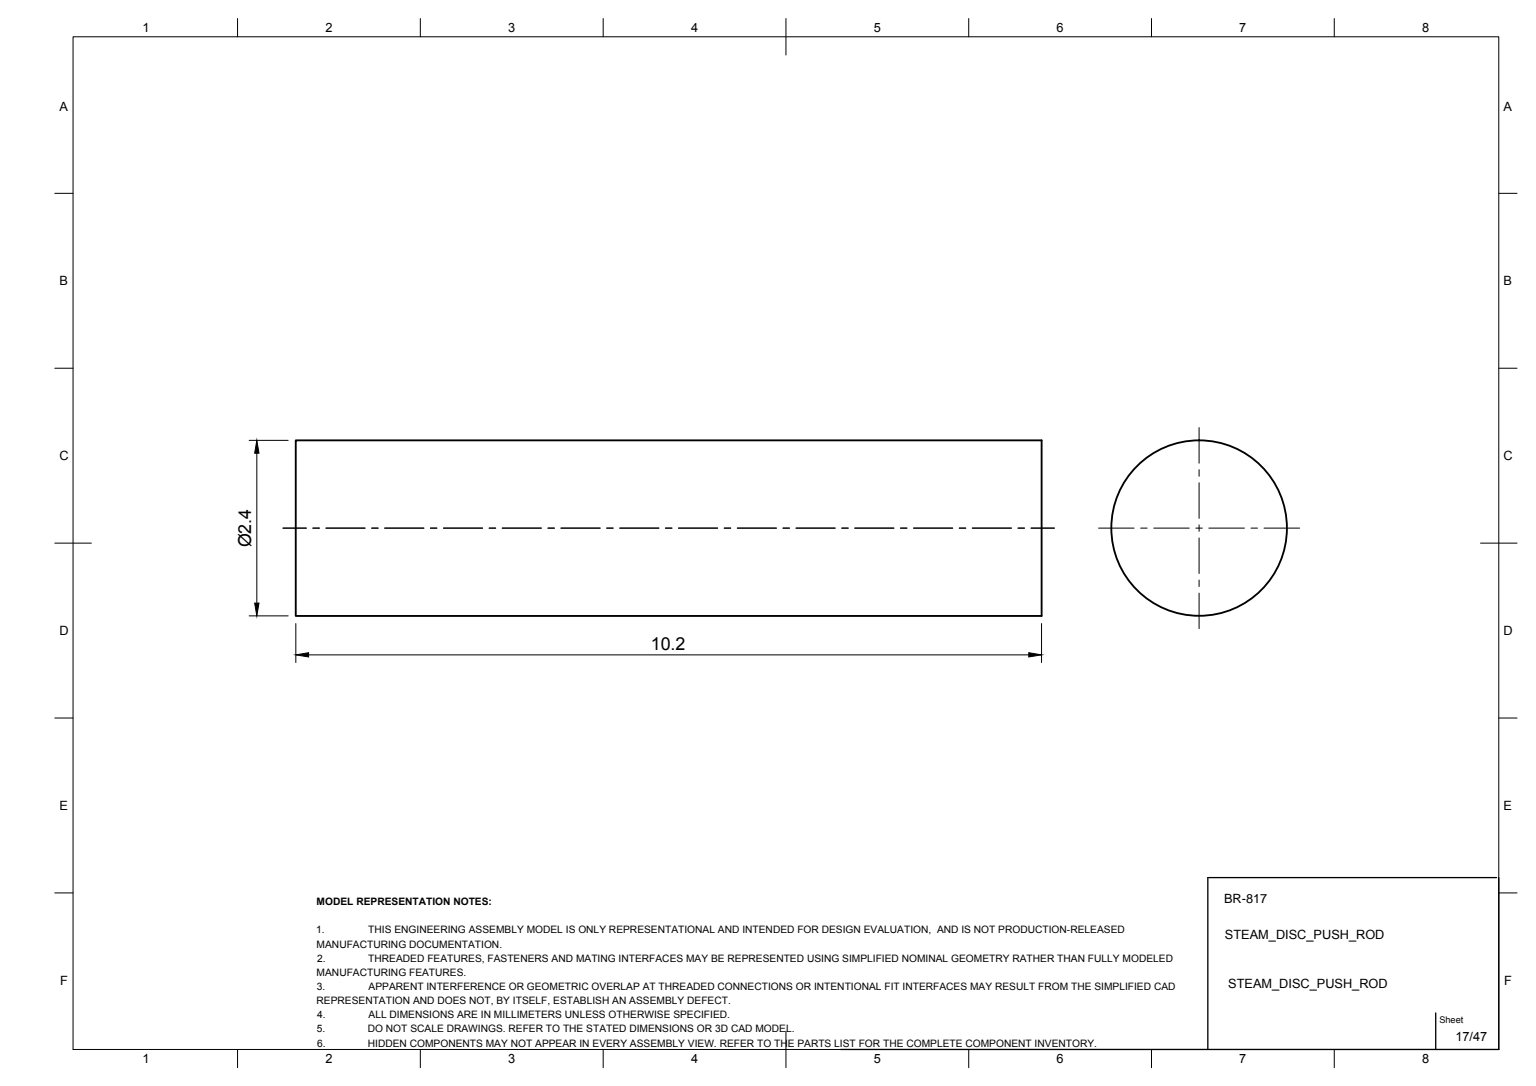
ISO-10303-21;
HEADER;
FILE_DESCRIPTION((''),'2;1');
FILE_NAME('STEAM_DISC_PUSH_ROD.step','2026-10-01T22:07:29-07:00',(''),(''),'','','');
FILE_SCHEMA (('AUTOMOTIVE_DESIGN { 1 0 10303 214 3 1 1 }'));
ENDSEC;
DATA;
#10=MECHANICAL_DESIGN_GEOMETRIC_PRESENTATION_REPRESENTATION('',(#551),#15484);
#481=SHAPE_REPRESENTATION_RELATIONSHIP('SRR','None',#15630,#516) ;
#516=ADVANCED_BREP_SHAPE_REPRESENTATION('',(#593),#15454) ;
#551=STYLED_ITEM('',(#15832),#593) ;
#593=MANIFOLD_SOLID_BREP('STEAM_DISC_PUSH_ROD',#8260) ;
#662=CYLINDRICAL_SURFACE('',#8894,0.12) ;
#958=CIRCLE('',#8895,0.12) ;
#959=CIRCLE('',#8896,0.12) ;
#1485=FACE_OUTER_BOUND('',#2028,.T.) ;
#1486=FACE_OUTER_BOUND('',#2029,.T.) ;
#1487=FACE_OUTER_BOUND('',#2030,.T.) ;
#2028=EDGE_LOOP('',(#5773,#5774,#5775,#5776)) ;
#2029=EDGE_LOOP('',(#5777)) ;
#2030=EDGE_LOOP('',(#5778)) ;
#2617=LINE('',#13445,#3091) ;
#3091=VECTOR('',#10530,0.12) ;
#3555=VERTEX_POINT('',#13442) ;
#3556=VERTEX_POINT('',#13444) ;
#4391=EDGE_CURVE('',#3555,#3555,#958,.T.) ;
#4392=EDGE_CURVE('',#3555,#3556,#2617,.T.) ;
#4393=EDGE_CURVE('',#3556,#3556,#959,.T.) ;
#5773=ORIENTED_EDGE('',*,*,#4391,.F.) ;
#5774=ORIENTED_EDGE('',*,*,#4392,.T.) ;
#5775=ORIENTED_EDGE('',*,*,#4393,.F.) ;
#5776=ORIENTED_EDGE('',*,*,#4392,.F.) ;
#5777=ORIENTED_EDGE('',*,*,#4393,.T.) ;
#5778=ORIENTED_EDGE('',*,*,#4391,.T.) ;
#7620=PLANE('',#8897) ;
#7621=PLANE('',#8898) ;
#7872=ADVANCED_FACE('',(#1485),#662,.T.) ;
#7873=ADVANCED_FACE('',(#1486),#7620,.T.) ;
#7874=ADVANCED_FACE('',(#1487),#7621,.T.) ;
#8260=CLOSED_SHELL('',(#7872,#7873,#7874)) ;
#8893=AXIS2_PLACEMENT_3D('',#13440,#10524,#10525) ;
#8894=AXIS2_PLACEMENT_3D('',#13441,#10526,#10527) ;
#8895=AXIS2_PLACEMENT_3D('',#13443,#10528,#10529) ;
#8896=AXIS2_PLACEMENT_3D('',#13446,#10531,#10532) ;
#8897=AXIS2_PLACEMENT_3D('',#13447,#10533,#10534) ;
#8898=AXIS2_PLACEMENT_3D('',#13448,#10535,#10536) ;
#10524=DIRECTION('axis',(0.,0.,1.)) ;
#10525=DIRECTION('refdir',(1.,0.,0.)) ;
#10526=DIRECTION('center_axis',(0.,0.,1.)) ;
#10527=DIRECTION('ref_axis',(1.,0.,0.)) ;
#10528=DIRECTION('center_axis',(0.,0.,1.)) ;
#10529=DIRECTION('ref_axis',(1.,0.,0.)) ;
#10530=DIRECTION('',(0.,0.,-1.)) ;
#10531=DIRECTION('center_axis',(0.,0.,-1.)) ;
#10532=DIRECTION('ref_axis',(1.,0.,0.)) ;
#10533=DIRECTION('center_axis',(0.,0.,-1.)) ;
#10534=DIRECTION('ref_axis',(-1.,0.,0.)) ;
#10535=DIRECTION('center_axis',(0.,0.,1.)) ;
#10536=DIRECTION('ref_axis',(1.,0.,0.)) ;
#13440=CARTESIAN_POINT('',(0.,0.,0.)) ;
#13441=CARTESIAN_POINT('Origin',(2.,0.8,1.64)) ;
#13442=CARTESIAN_POINT('',(1.88,0.8,2.15)) ;
#13443=CARTESIAN_POINT('Origin',(2.,0.8,2.15)) ;
#13444=CARTESIAN_POINT('',(1.88,0.8,1.13)) ;
#13445=CARTESIAN_POINT('',(1.88,0.8,1.64)) ;
#13446=CARTESIAN_POINT('Origin',(2.,0.8,1.13)) ;
#13447=CARTESIAN_POINT('Origin',(2.,0.8,1.13)) ;
#13448=CARTESIAN_POINT('Origin',(2.,0.8,2.15)) ;
#15411=UNCERTAINTY_MEASURE_WITH_UNIT(LENGTH_MEASURE(0.001),#15485,
'DISTANCE_ACCURACY_VALUE',
'Maximum model space distance between geometric entities at asserted c
onnectivities') ;
#15441=UNCERTAINTY_MEASURE_WITH_UNIT(LENGTH_MEASURE(0.001),#15485,
'DISTANCE_ACCURACY_VALUE',
'Maximum model space distance between geometric entities at asserted c
onnectivities') ;
#15454=(
GEOMETRIC_REPRESENTATION_CONTEXT(3)
GLOBAL_UNCERTAINTY_ASSIGNED_CONTEXT((#15411))
GLOBAL_UNIT_ASSIGNED_CONTEXT((#15485,#15487,#15488))
REPRESENTATION_CONTEXT('','3D')
) ;
#15484=(
GEOMETRIC_REPRESENTATION_CONTEXT(3)
GLOBAL_UNCERTAINTY_ASSIGNED_CONTEXT((#15441))
GLOBAL_UNIT_ASSIGNED_CONTEXT((#15485,#15487,#15488))
REPRESENTATION_CONTEXT('','3D')
) ;
#15485=(
LENGTH_UNIT()
NAMED_UNIT(*)
SI_UNIT(.CENTI.,.METRE.)
) ;
#15487=(
NAMED_UNIT(*)
PLANE_ANGLE_UNIT()
SI_UNIT($,.RADIAN.)
) ;
#15488=(
NAMED_UNIT(*)
SI_UNIT($,.STERADIAN.)
SOLID_ANGLE_UNIT()
) ;
#15501=SHAPE_DEFINITION_REPRESENTATION(#15549,#15630) ;
#15549=PRODUCT_DEFINITION_SHAPE('',$,#15673) ;
#15630=SHAPE_REPRESENTATION('',(#8893),#15454) ;
#15660=PRODUCT_DEFINITION_CONTEXT('part definition',#15788,'design') ;
#15673=PRODUCT_DEFINITION('STEAM_DISC_PUSH_ROD',
'STEAM_DISC_PUSH_ROD',#15715,#15660) ;
#15715=PRODUCT_DEFINITION_FORMATION('',$,#15802) ;
#15788=APPLICATION_CONTEXT(
'Core Data for Automotive Mechanical Design Process') ;
#15789=PRODUCT_CONTEXT('part definition',#15788,'mechanical') ;
#15802=PRODUCT('STEAM_DISC_PUSH_ROD','STEAM_DISC_PUSH_ROD',$,(#15789)) ;
#15832=PRESENTATION_STYLE_ASSIGNMENT((#15844)) ;
#15844=SURFACE_STYLE_USAGE(.BOTH.,#15856) ;
#15856=SURFACE_SIDE_STYLE('',(#15868)) ;
#15868=SURFACE_STYLE_FILL_AREA(#15880) ;
#15880=FILL_AREA_STYLE('Steel - Satin',(#15892)) ;
#15892=FILL_AREA_STYLE_COLOUR('Steel - Satin',#15904) ;
#15904=COLOUR_RGB('Steel - Satin', 0.72549020, 0.75294118, 0.79215686) ;
ENDSEC;
END-ISO-10303-21;
